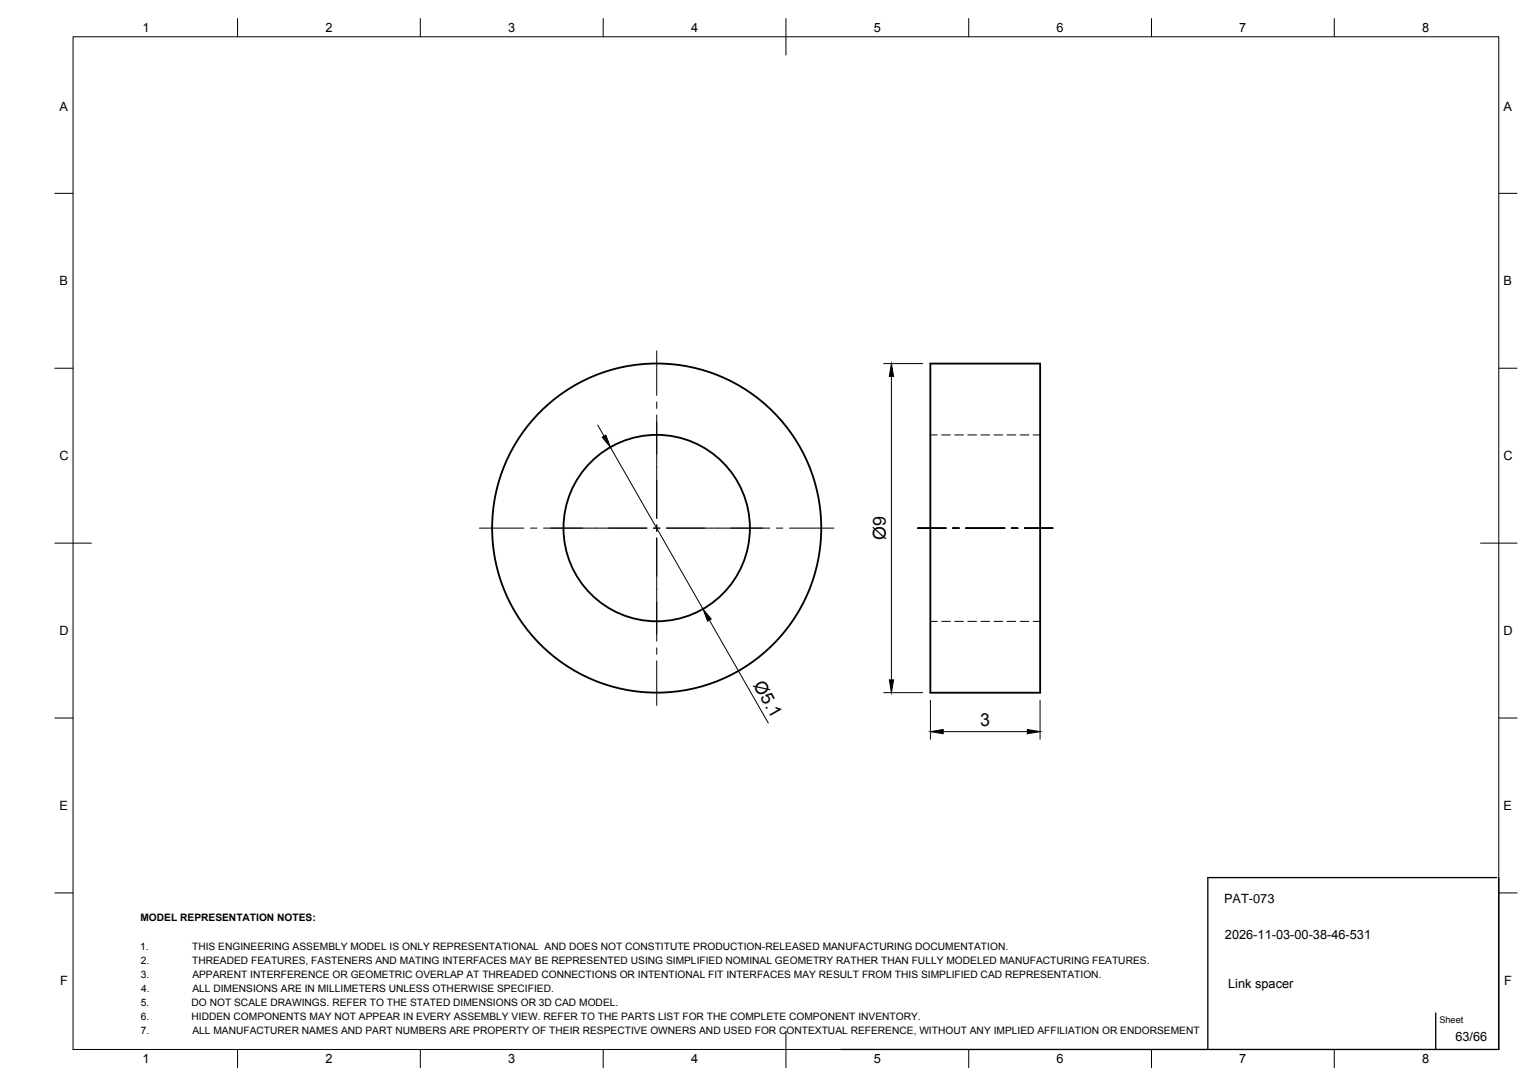
ISO-10303-21;
HEADER;
/* Generated by software containing ST-Developer
 * from STEP Tools, Inc. (www.steptools.com) 
 */

FILE_DESCRIPTION(
/* description */ ('Manual piston pump'),
/* implementation_level */ '2;1');

FILE_NAME(
/* name */ 'Link spacer.step',
/* time_stamp */ '2026-11-02T16:54:23-08:00',
/* author */ (''),
/* organization */ (''),
/* preprocessor_version */ 'ST-DEVELOPER v20.2',
/* originating_system */ 'Autodesk Translation Framework v15.17.0.0',
/* authorisation */ '');

FILE_SCHEMA (('AUTOMOTIVE_DESIGN { 1 0 10303 214 3 1 1 }'));
ENDSEC;

DATA;
#10=MECHANICAL_DESIGN_GEOMETRIC_PRESENTATION_REPRESENTATION('',(#755),#19043);
#620=SHAPE_REPRESENTATION_RELATIONSHIP('SRR','None',#19370,#683);
#683=ADVANCED_BREP_SHAPE_REPRESENTATION('',(#823),#19037);
#755=STYLED_ITEM('',(#19664),#823);
#823=MANIFOLD_SOLID_BREP('Body1',#9543);
#1037=FACE_BOUND('',#2619,.T.);
#1038=FACE_BOUND('',#2621,.T.);
#1280=CYLINDRICAL_SURFACE('',#11396,0.255000000000001);
#1281=CYLINDRICAL_SURFACE('',#11399,0.449999999999999);
#1831=FACE_OUTER_BOUND('',#2616,.T.);
#1832=FACE_OUTER_BOUND('',#2617,.T.);
#1833=FACE_OUTER_BOUND('',#2618,.T.);
#1834=FACE_OUTER_BOUND('',#2620,.T.);
#2616=EDGE_LOOP('',(#8441,#8442,#8443,#8444));
#2617=EDGE_LOOP('',(#8445,#8446,#8447,#8448));
#2618=EDGE_LOOP('',(#8449));
#2619=EDGE_LOOP('',(#8450));
#2620=EDGE_LOOP('',(#8451));
#2621=EDGE_LOOP('',(#8452));
#3120=CIRCLE('',#11397,0.255000000000001);
#3121=CIRCLE('',#11398,0.255000000000001);
#3122=CIRCLE('',#11400,0.449999999999999);
#3123=CIRCLE('',#11401,0.449999999999999);
#3712=LINE('',#18725,#4316);
#3713=LINE('',#18731,#4317);
#4316=VECTOR('',#14370,0.255000000000001);
#4317=VECTOR('',#14377,0.449999999999999);
#5080=VERTEX_POINT('',#18722);
#5081=VERTEX_POINT('',#18724);
#5082=VERTEX_POINT('',#18728);
#5083=VERTEX_POINT('',#18730);
#6207=EDGE_CURVE('',#5080,#5080,#3120,.T.);
#6208=EDGE_CURVE('',#5080,#5081,#3712,.T.);
#6209=EDGE_CURVE('',#5081,#5081,#3121,.T.);
#6210=EDGE_CURVE('',#5082,#5082,#3122,.T.);
#6211=EDGE_CURVE('',#5082,#5083,#3713,.T.);
#6212=EDGE_CURVE('',#5083,#5083,#3123,.T.);
#8441=ORIENTED_EDGE('',*,*,#6207,.F.);
#8442=ORIENTED_EDGE('',*,*,#6208,.T.);
#8443=ORIENTED_EDGE('',*,*,#6209,.T.);
#8444=ORIENTED_EDGE('',*,*,#6208,.F.);
#8445=ORIENTED_EDGE('',*,*,#6210,.F.);
#8446=ORIENTED_EDGE('',*,*,#6211,.T.);
#8447=ORIENTED_EDGE('',*,*,#6212,.T.);
#8448=ORIENTED_EDGE('',*,*,#6211,.F.);
#8449=ORIENTED_EDGE('',*,*,#6210,.T.);
#8450=ORIENTED_EDGE('',*,*,#6207,.T.);
#8451=ORIENTED_EDGE('',*,*,#6212,.F.);
#8452=ORIENTED_EDGE('',*,*,#6209,.F.);
#8876=PLANE('',#11402);
#8877=PLANE('',#11403);
#9436=ADVANCED_FACE('',(#1831),#1280,.F.);
#9437=ADVANCED_FACE('',(#1832),#1281,.T.);
#9438=ADVANCED_FACE('',(#1833,#1037),#8876,.T.);
#9439=ADVANCED_FACE('',(#1834,#1038),#8877,.F.);
#9543=CLOSED_SHELL('',(#9436,#9437,#9438,#9439));
#11395=AXIS2_PLACEMENT_3D('',#18720,#14364,#14365);
#11396=AXIS2_PLACEMENT_3D('',#18721,#14366,#14367);
#11397=AXIS2_PLACEMENT_3D('',#18723,#14368,#14369);
#11398=AXIS2_PLACEMENT_3D('',#18726,#14371,#14372);
#11399=AXIS2_PLACEMENT_3D('',#18727,#14373,#14374);
#11400=AXIS2_PLACEMENT_3D('',#18729,#14375,#14376);
#11401=AXIS2_PLACEMENT_3D('',#18732,#14378,#14379);
#11402=AXIS2_PLACEMENT_3D('',#18733,#14380,#14381);
#11403=AXIS2_PLACEMENT_3D('',#18734,#14382,#14383);
#14364=DIRECTION('axis',(0.,0.,1.));
#14365=DIRECTION('refdir',(1.,0.,0.));
#14366=DIRECTION('center_axis',(1.,0.,0.));
#14367=DIRECTION('ref_axis',(0.,0.,-1.));
#14368=DIRECTION('center_axis',(-1.,0.,0.));
#14369=DIRECTION('ref_axis',(0.,0.,-1.));
#14370=DIRECTION('',(-1.,0.,0.));
#14371=DIRECTION('center_axis',(-1.,0.,0.));
#14372=DIRECTION('ref_axis',(0.,0.,-1.));
#14373=DIRECTION('center_axis',(1.,0.,0.));
#14374=DIRECTION('ref_axis',(0.,0.,-1.));
#14375=DIRECTION('center_axis',(1.,0.,0.));
#14376=DIRECTION('ref_axis',(0.,0.,-1.));
#14377=DIRECTION('',(-1.,0.,0.));
#14378=DIRECTION('center_axis',(1.,0.,0.));
#14379=DIRECTION('ref_axis',(0.,0.,-1.));
#14380=DIRECTION('center_axis',(1.,0.,0.));
#14381=DIRECTION('ref_axis',(0.,0.,-1.));
#14382=DIRECTION('center_axis',(1.,0.,0.));
#14383=DIRECTION('ref_axis',(0.,0.,-1.));
#18720=CARTESIAN_POINT('',(0.,0.,0.));
#18721=CARTESIAN_POINT('Origin',(-0.6,-8.,10.));
#18722=CARTESIAN_POINT('',(-0.3,-8.,10.255));
#18723=CARTESIAN_POINT('Origin',(-0.3,-8.,10.));
#18724=CARTESIAN_POINT('',(-0.6,-8.,10.255));
#18725=CARTESIAN_POINT('',(-0.6,-8.,10.255));
#18726=CARTESIAN_POINT('Origin',(-0.6,-8.,10.));
#18727=CARTESIAN_POINT('Origin',(-0.6,-8.,10.));
#18728=CARTESIAN_POINT('',(-0.3,-8.,10.45));
#18729=CARTESIAN_POINT('Origin',(-0.3,-8.,10.));
#18730=CARTESIAN_POINT('',(-0.6,-8.,10.45));
#18731=CARTESIAN_POINT('',(-0.6,-8.,10.45));
#18732=CARTESIAN_POINT('Origin',(-0.6,-8.,10.));
#18733=CARTESIAN_POINT('Origin',(-0.3,-8.,10.));
#18734=CARTESIAN_POINT('Origin',(-0.6,-8.,10.));
#18966=UNCERTAINTY_MEASURE_WITH_UNIT(LENGTH_MEASURE(0.001),#19044,
'DISTANCE_ACCURACY_VALUE',
'Maximum model space distance between geometric entities at asserted c
onnectivities');
#18972=UNCERTAINTY_MEASURE_WITH_UNIT(LENGTH_MEASURE(0.001),#19044,
'DISTANCE_ACCURACY_VALUE',
'Maximum model space distance between geometric entities at asserted c
onnectivities');
#19037=(
GEOMETRIC_REPRESENTATION_CONTEXT(3)
GLOBAL_UNCERTAINTY_ASSIGNED_CONTEXT((#18966))
GLOBAL_UNIT_ASSIGNED_CONTEXT((#19044,#19046,#19047))
REPRESENTATION_CONTEXT('','3D')
);
#19043=(
GEOMETRIC_REPRESENTATION_CONTEXT(3)
GLOBAL_UNCERTAINTY_ASSIGNED_CONTEXT((#18972))
GLOBAL_UNIT_ASSIGNED_CONTEXT((#19044,#19046,#19047))
REPRESENTATION_CONTEXT('','3D')
);
#19044=(
LENGTH_UNIT()
NAMED_UNIT(*)
SI_UNIT(.CENTI.,.METRE.)
);
#19046=(
NAMED_UNIT(*)
PLANE_ANGLE_UNIT()
SI_UNIT($,.RADIAN.)
);
#19047=(
NAMED_UNIT(*)
SI_UNIT($,.STERADIAN.)
SOLID_ANGLE_UNIT()
);
#19112=SHAPE_DEFINITION_REPRESENTATION(#19269,#19370);
#19269=PRODUCT_DEFINITION_SHAPE('',$,#19441);
#19370=SHAPE_REPRESENTATION('',(#11395),#19037);
#19376=PRODUCT_DEFINITION_CONTEXT('part definition',#19588,'design');
#19441=PRODUCT_DEFINITION('2026-11-03-00-38-46-531','Link spacer',#19511,
#19376);
#19511=PRODUCT_DEFINITION_FORMATION('',$,#19654);
#19588=APPLICATION_CONTEXT(
'Core Data for Automotive Mechanical Design Process');
#19589=PRODUCT_CONTEXT('part definition',#19588,'mechanical');
#19654=PRODUCT('2026-11-03-00-38-46-531','Link spacer','Link spacer',(#19589));
#19664=PRESENTATION_STYLE_ASSIGNMENT((#19670));
#19670=SURFACE_STYLE_USAGE(.BOTH.,#19676);
#19676=SURFACE_SIDE_STYLE('',(#19682));
#19682=SURFACE_STYLE_FILL_AREA(#19688);
#19688=FILL_AREA_STYLE('CAD Library Painted - Steel gray',(#19694));
#19694=FILL_AREA_STYLE_COLOUR('CAD Library Painted - Steel gray',#19700);
#19700=COLOUR_RGB('CAD Library Painted - Steel gray',0.592156862745098,
0.631372549019608,0.67843137254902);
ENDSEC;
END-ISO-10303-21;
